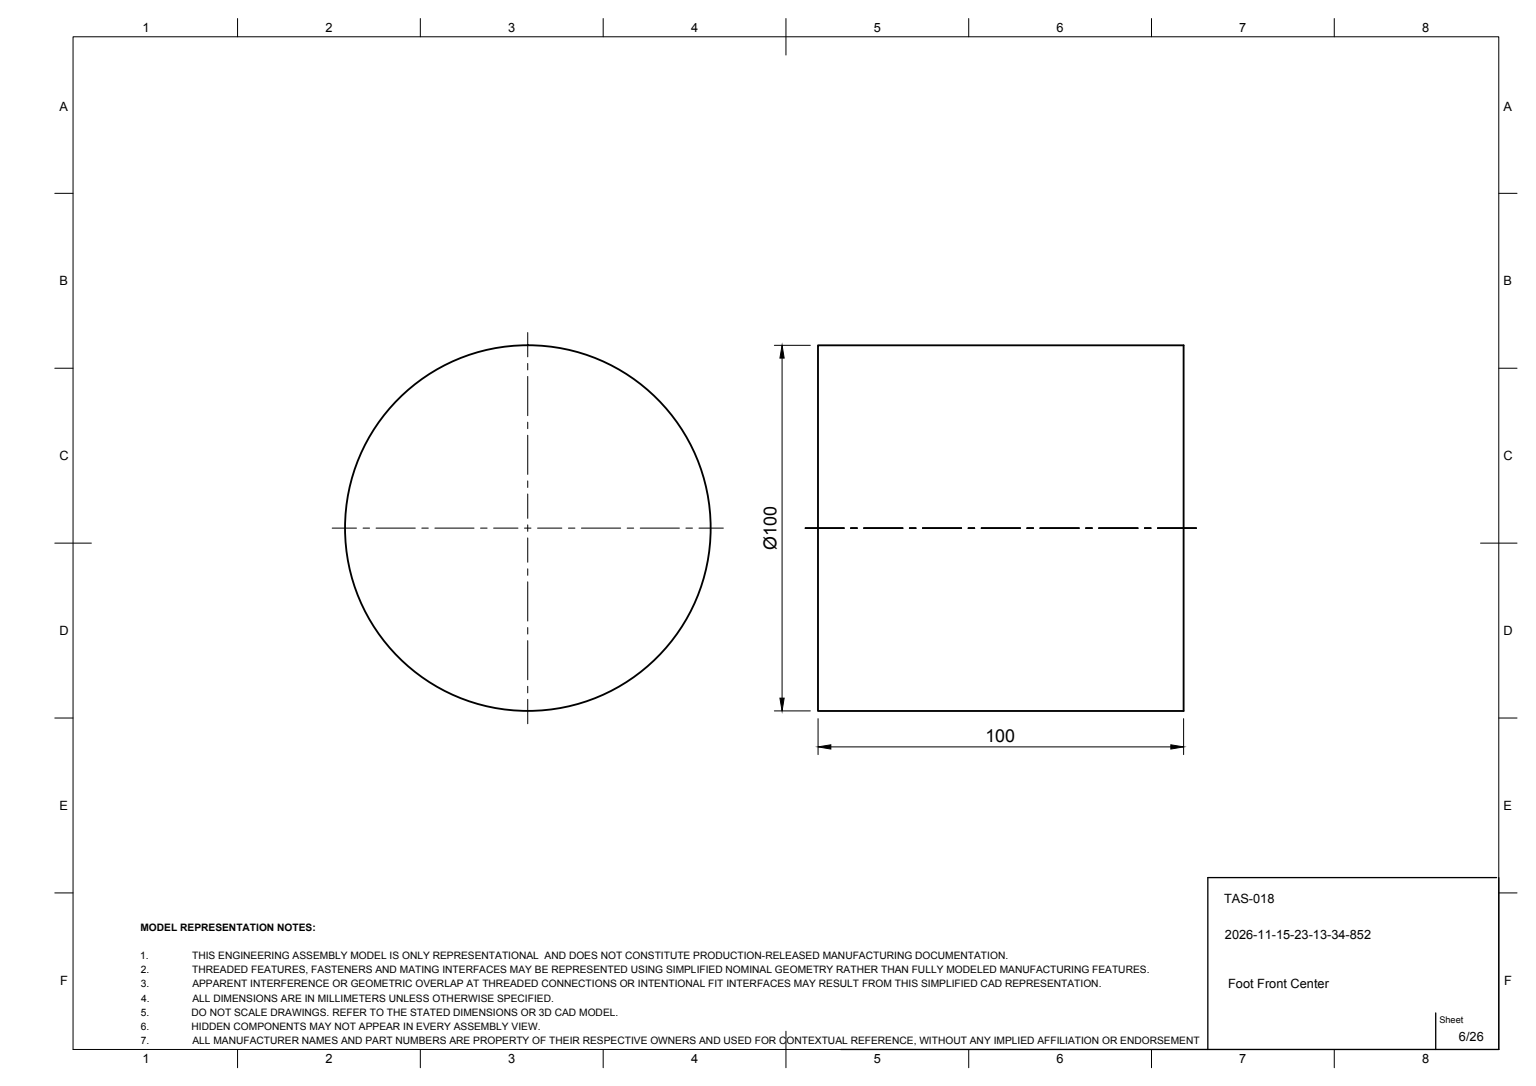
ISO-10303-21;
HEADER;
/* Generated by software containing ST-Developer
 * from STEP Tools, Inc. (www.steptools.com) 
 */

FILE_DESCRIPTION(
/* description */ (''),
/* implementation_level */ '2;1');

FILE_NAME(
/* name */ 'Foot Front Center.step',
/* time_stamp */ '2026-11-15T15:17:57-08:00',
/* author */ (''),
/* organization */ (''),
/* preprocessor_version */ 'ST-DEVELOPER v20.2',
/* originating_system */ 'Autodesk Translation Framework v15.17.0.0',
/* authorisation */ '');

FILE_SCHEMA (('AUTOMOTIVE_DESIGN { 1 0 10303 214 3 1 1 }'));
ENDSEC;

DATA;
#10=MECHANICAL_DESIGN_GEOMETRIC_PRESENTATION_REPRESENTATION('',(#181),#3723);
#11=CIRCLE('',#2347,1.96850393700787);
#12=CIRCLE('',#2348,1.96850393700787);
#23=CYLINDRICAL_SURFACE('',#2346,1.96850393700787);
#133=SHAPE_REPRESENTATION_RELATIONSHIP('SRR','None',#3814,#157);
#157=ADVANCED_BREP_SHAPE_REPRESENTATION('',(#205),#3703);
#181=STYLED_ITEM('',(#3945),#205);
#205=MANIFOLD_SOLID_BREP('Body1',#2029);
#249=FACE_OUTER_BOUND('',#375,.T.);
#250=FACE_OUTER_BOUND('',#376,.T.);
#251=FACE_OUTER_BOUND('',#377,.T.);
#375=EDGE_LOOP('',(#1407,#1408,#1409,#1410));
#376=EDGE_LOOP('',(#1411));
#377=EDGE_LOOP('',(#1412));
#525=LINE('',#3219,#747);
#747=VECTOR('',#2619,1.96850393700787);
#953=VERTEX_POINT('',#3216);
#954=VERTEX_POINT('',#3218);
#1125=EDGE_CURVE('',#953,#953,#11,.T.);
#1126=EDGE_CURVE('',#953,#954,#525,.T.);
#1127=EDGE_CURVE('',#954,#954,#12,.T.);
#1407=ORIENTED_EDGE('',*,*,#1125,.T.);
#1408=ORIENTED_EDGE('',*,*,#1126,.T.);
#1409=ORIENTED_EDGE('',*,*,#1127,.F.);
#1410=ORIENTED_EDGE('',*,*,#1126,.F.);
#1411=ORIENTED_EDGE('',*,*,#1127,.T.);
#1412=ORIENTED_EDGE('',*,*,#1125,.F.);
#1803=PLANE('',#2349);
#1804=PLANE('',#2350);
#1923=ADVANCED_FACE('',(#249),#23,.T.);
#1924=ADVANCED_FACE('',(#250),#1803,.T.);
#1925=ADVANCED_FACE('',(#251),#1804,.F.);
#2029=CLOSED_SHELL('',(#1923,#1924,#1925));
#2345=AXIS2_PLACEMENT_3D('',#3214,#2613,#2614);
#2346=AXIS2_PLACEMENT_3D('',#3215,#2615,#2616);
#2347=AXIS2_PLACEMENT_3D('',#3217,#2617,#2618);
#2348=AXIS2_PLACEMENT_3D('',#3220,#2620,#2621);
#2349=AXIS2_PLACEMENT_3D('',#3221,#2622,#2623);
#2350=AXIS2_PLACEMENT_3D('',#3222,#2624,#2625);
#2613=DIRECTION('axis',(0.,0.,1.));
#2614=DIRECTION('refdir',(1.,0.,0.));
#2615=DIRECTION('center_axis',(0.,1.,0.));
#2616=DIRECTION('ref_axis',(0.,0.,1.));
#2617=DIRECTION('center_axis',(0.,-1.,0.));
#2618=DIRECTION('ref_axis',(0.,0.,-1.));
#2619=DIRECTION('',(0.,-1.,0.));
#2620=DIRECTION('center_axis',(0.,-1.,0.));
#2621=DIRECTION('ref_axis',(0.,0.,-1.));
#2622=DIRECTION('center_axis',(0.,-1.,0.));
#2623=DIRECTION('ref_axis',(0.,0.,-1.));
#2624=DIRECTION('center_axis',(0.,-1.,0.));
#2625=DIRECTION('ref_axis',(0.,0.,-1.));
#3214=CARTESIAN_POINT('',(0.,0.,0.));
#3215=CARTESIAN_POINT('Origin',(8.74191357972564E-15,-4.91732638859567E-15,
19.6377952755906));
#3216=CARTESIAN_POINT('',(8.74191357972564E-15,3.93700787401574,17.6692913385827));
#3217=CARTESIAN_POINT('Origin',(8.74191357972564E-15,3.93700787401574,19.6377952755906));
#3218=CARTESIAN_POINT('',(8.74191357972564E-15,-4.91732638859567E-15,17.6692913385827));
#3219=CARTESIAN_POINT('',(8.50084137516908E-15,-4.91732638859567E-15,17.6692913385827));
#3220=CARTESIAN_POINT('Origin',(8.74191357972564E-15,-4.91732638859567E-15,
19.6377952755906));
#3221=CARTESIAN_POINT('Origin',(8.74191357972564E-15,-4.91732638859567E-15,
19.6377952755906));
#3222=CARTESIAN_POINT('Origin',(8.74191357972564E-15,3.93700787401574,19.6377952755906));
#3676=UNCERTAINTY_MEASURE_WITH_UNIT(LENGTH_MEASURE(0.000393700787401575),
#3725,'DISTANCE_ACCURACY_VALUE',
'Maximum model space distance between geometric entities at asserted c
onnectivities');
#3696=UNCERTAINTY_MEASURE_WITH_UNIT(LENGTH_MEASURE(0.000393700787401575),
#3725,'DISTANCE_ACCURACY_VALUE',
'Maximum model space distance between geometric entities at asserted c
onnectivities');
#3703=(
GEOMETRIC_REPRESENTATION_CONTEXT(3)
GLOBAL_UNCERTAINTY_ASSIGNED_CONTEXT((#3676))
GLOBAL_UNIT_ASSIGNED_CONTEXT((#3725,#3729,#3730))
REPRESENTATION_CONTEXT('','3D')
);
#3723=(
GEOMETRIC_REPRESENTATION_CONTEXT(3)
GLOBAL_UNCERTAINTY_ASSIGNED_CONTEXT((#3696))
GLOBAL_UNIT_ASSIGNED_CONTEXT((#3725,#3729,#3730))
REPRESENTATION_CONTEXT('','3D')
);
#3724=DIMENSIONAL_EXPONENTS(1.,0.,0.,0.,0.,0.,0.);
#3725=(
CONVERSION_BASED_UNIT('inch',#3728)
LENGTH_UNIT()
NAMED_UNIT(#3724)
);
#3726=(
LENGTH_UNIT()
NAMED_UNIT(*)
SI_UNIT(.MILLI.,.METRE.)
);
#3728=LENGTH_MEASURE_WITH_UNIT(LENGTH_MEASURE(25.4),#3726);
#3729=(
NAMED_UNIT(*)
PLANE_ANGLE_UNIT()
SI_UNIT($,.RADIAN.)
);
#3730=(
NAMED_UNIT(*)
SI_UNIT($,.STERADIAN.)
SOLID_ANGLE_UNIT()
);
#3737=SHAPE_DEFINITION_REPRESENTATION(#3764,#3814);
#3764=PRODUCT_DEFINITION_SHAPE('',$,#3841);
#3814=SHAPE_REPRESENTATION('',(#2345),#3703);
#3834=PRODUCT_DEFINITION_CONTEXT('part definition',#3914,'design');
#3841=PRODUCT_DEFINITION('2026-11-15-23-13-34-852','Foot Front Center',
#3867,#3834);
#3867=PRODUCT_DEFINITION_FORMATION('',$,#3922);
#3914=APPLICATION_CONTEXT(
'Core Data for Automotive Mechanical Design Process');
#3915=PRODUCT_CONTEXT('part definition',#3914,'mechanical');
#3922=PRODUCT('2026-11-15-23-13-34-852','Foot Front Center',$,(#3915));
#3945=PRESENTATION_STYLE_ASSIGNMENT((#3953));
#3953=SURFACE_STYLE_USAGE(.BOTH.,#3961);
#3961=SURFACE_SIDE_STYLE('',(#3969));
#3969=SURFACE_STYLE_FILL_AREA(#3977);
#3977=FILL_AREA_STYLE('Black',(#3985));
#3985=FILL_AREA_STYLE_COLOUR('Black',#3993);
#3993=COLOUR_RGB('Black',0.0784313725490196,0.0784313725490196,0.0784313725490196);
ENDSEC;
END-ISO-10303-21;
